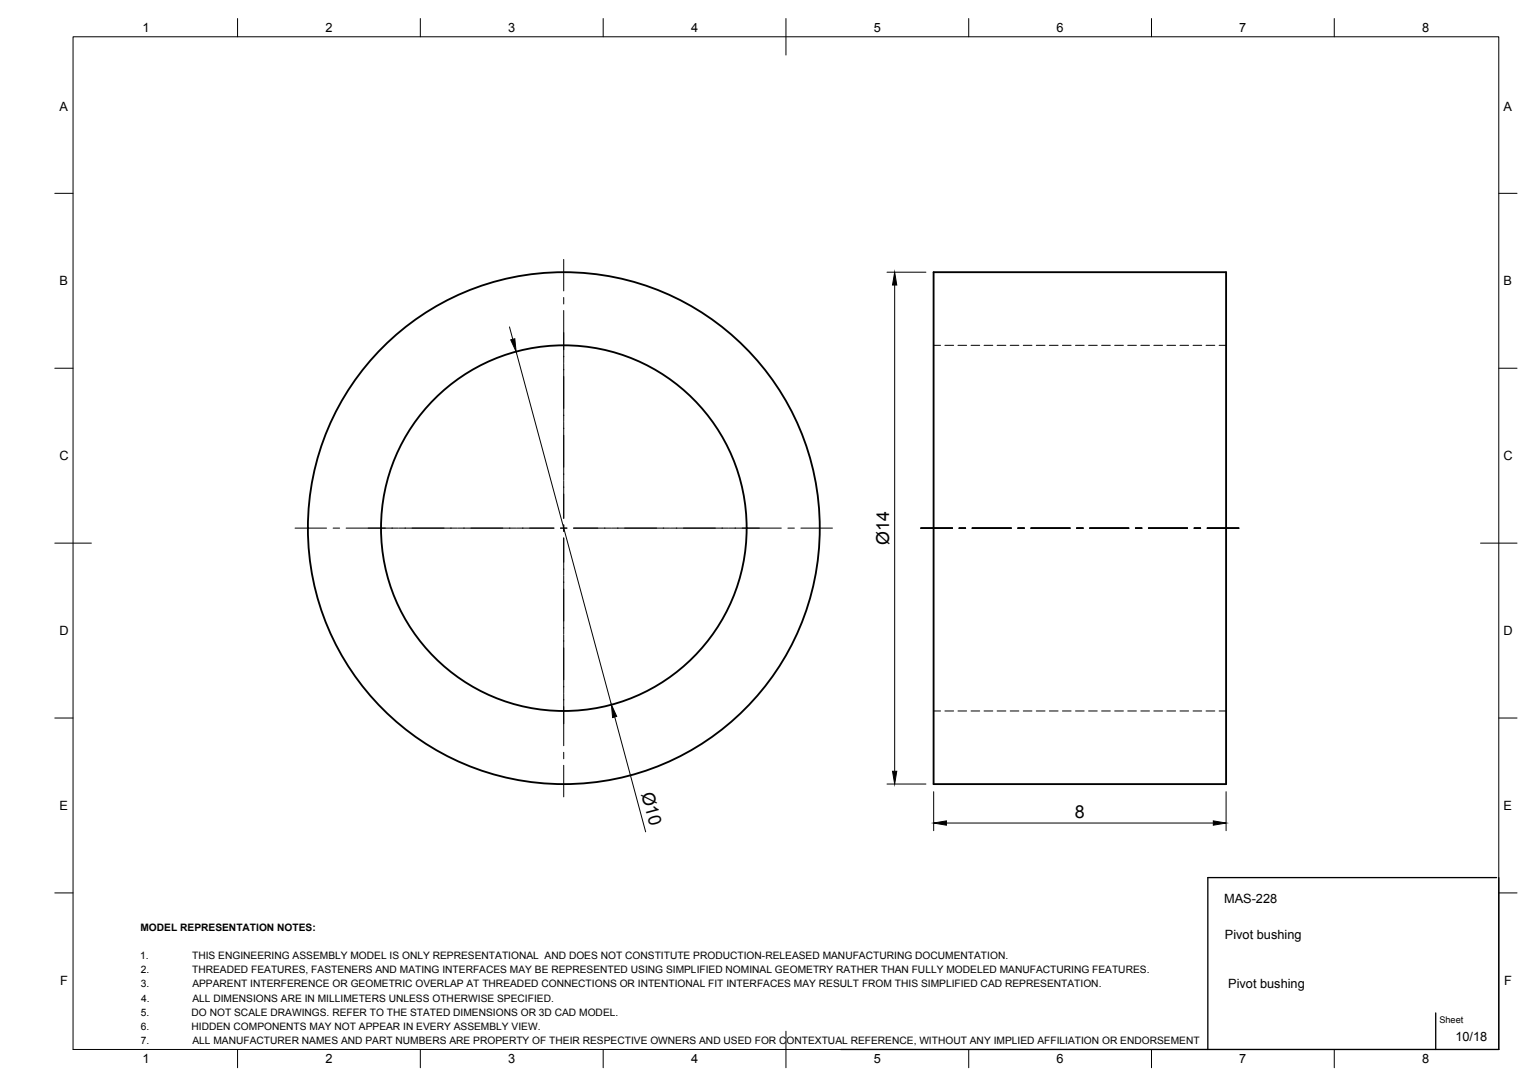
ISO-10303-21;
HEADER;
/* Generated by software containing ST-Developer
 * from STEP Tools, Inc. (www.steptools.com) 
 */

FILE_DESCRIPTION(
/* description */ ('Independent Peaucellier-Lipkin straight-line linkage. Radius arms 100
 mm, inversion-cell links 60 mm, crank radius and fixed-pivot spacing 
32 mm. Inversion constant 6400 mm squared, nominal output straight lin
e X=100 mm. Overhead bearing bridge clears the layered moving links. N
o accuracy or load rating assigned.'),
/* implementation_level */ '2;1');

FILE_NAME(
/* name */ 'Pivot bushing.step',
/* time_stamp */ '2026-11-09T18:06:16-08:00',
/* author */ (''),
/* organization */ (''),
/* preprocessor_version */ 'ST-DEVELOPER v20.2',
/* originating_system */ 'Autodesk Translation Framework v15.17.0.0',
/* authorisation */ '');

FILE_SCHEMA (('AUTOMOTIVE_DESIGN { 1 0 10303 214 3 1 1 }'));
ENDSEC;

DATA;
#10=MECHANICAL_DESIGN_GEOMETRIC_PRESENTATION_REPRESENTATION('',(#293),#3581);
#259=SHAPE_REPRESENTATION_RELATIONSHIP('SRR','None',#3693,#276);
#276=ADVANCED_BREP_SHAPE_REPRESENTATION('',(#310),#3575);
#293=STYLED_ITEM('',(#3784),#310);
#310=MANIFOLD_SOLID_BREP('Body1',#1879);
#355=FACE_BOUND('',#659,.T.);
#356=FACE_BOUND('',#661,.T.);
#409=PLANE('',#2245);
#410=PLANE('',#2246);
#506=FACE_OUTER_BOUND('',#656,.T.);
#507=FACE_OUTER_BOUND('',#657,.T.);
#508=FACE_OUTER_BOUND('',#658,.T.);
#509=FACE_OUTER_BOUND('',#660,.T.);
#656=EDGE_LOOP('',(#1616,#1617,#1618,#1619));
#657=EDGE_LOOP('',(#1620,#1621,#1622,#1623));
#658=EDGE_LOOP('',(#1624));
#659=EDGE_LOOP('',(#1625));
#660=EDGE_LOOP('',(#1626));
#661=EDGE_LOOP('',(#1627));
#773=LINE('',#3377,#871);
#774=LINE('',#3383,#872);
#871=VECTOR('',#2773,5.);
#872=VECTOR('',#2780,7.);
#963=CIRCLE('',#2240,5.);
#964=CIRCLE('',#2241,5.);
#965=CIRCLE('',#2243,7.);
#966=CIRCLE('',#2244,7.);
#1089=VERTEX_POINT('',#3374);
#1090=VERTEX_POINT('',#3376);
#1091=VERTEX_POINT('',#3380);
#1092=VERTEX_POINT('',#3382);
#1270=EDGE_CURVE('',#1089,#1089,#963,.T.);
#1271=EDGE_CURVE('',#1089,#1090,#773,.T.);
#1272=EDGE_CURVE('',#1090,#1090,#964,.T.);
#1273=EDGE_CURVE('',#1091,#1091,#965,.T.);
#1274=EDGE_CURVE('',#1091,#1092,#774,.T.);
#1275=EDGE_CURVE('',#1092,#1092,#966,.T.);
#1616=ORIENTED_EDGE('',*,*,#1270,.F.);
#1617=ORIENTED_EDGE('',*,*,#1271,.T.);
#1618=ORIENTED_EDGE('',*,*,#1272,.T.);
#1619=ORIENTED_EDGE('',*,*,#1271,.F.);
#1620=ORIENTED_EDGE('',*,*,#1273,.F.);
#1621=ORIENTED_EDGE('',*,*,#1274,.T.);
#1622=ORIENTED_EDGE('',*,*,#1275,.T.);
#1623=ORIENTED_EDGE('',*,*,#1274,.F.);
#1624=ORIENTED_EDGE('',*,*,#1273,.T.);
#1625=ORIENTED_EDGE('',*,*,#1270,.T.);
#1626=ORIENTED_EDGE('',*,*,#1275,.F.);
#1627=ORIENTED_EDGE('',*,*,#1272,.F.);
#1744=CYLINDRICAL_SURFACE('',#2239,5.);
#1745=CYLINDRICAL_SURFACE('',#2242,7.);
#1838=ADVANCED_FACE('',(#506),#1744,.F.);
#1839=ADVANCED_FACE('',(#507),#1745,.T.);
#1840=ADVANCED_FACE('',(#508,#355),#409,.T.);
#1841=ADVANCED_FACE('',(#509,#356),#410,.F.);
#1879=CLOSED_SHELL('',(#1838,#1839,#1840,#1841));
#2238=AXIS2_PLACEMENT_3D('',#3372,#2767,#2768);
#2239=AXIS2_PLACEMENT_3D('',#3373,#2769,#2770);
#2240=AXIS2_PLACEMENT_3D('',#3375,#2771,#2772);
#2241=AXIS2_PLACEMENT_3D('',#3378,#2774,#2775);
#2242=AXIS2_PLACEMENT_3D('',#3379,#2776,#2777);
#2243=AXIS2_PLACEMENT_3D('',#3381,#2778,#2779);
#2244=AXIS2_PLACEMENT_3D('',#3384,#2781,#2782);
#2245=AXIS2_PLACEMENT_3D('',#3385,#2783,#2784);
#2246=AXIS2_PLACEMENT_3D('',#3386,#2785,#2786);
#2767=DIRECTION('axis',(0.,0.,1.));
#2768=DIRECTION('refdir',(1.,0.,0.));
#2769=DIRECTION('center_axis',(0.,0.,1.));
#2770=DIRECTION('ref_axis',(1.,0.,0.));
#2771=DIRECTION('center_axis',(0.,0.,-1.));
#2772=DIRECTION('ref_axis',(1.,0.,0.));
#2773=DIRECTION('',(0.,0.,-1.));
#2774=DIRECTION('center_axis',(0.,0.,-1.));
#2775=DIRECTION('ref_axis',(1.,0.,0.));
#2776=DIRECTION('center_axis',(0.,0.,1.));
#2777=DIRECTION('ref_axis',(1.,0.,0.));
#2778=DIRECTION('center_axis',(0.,0.,1.));
#2779=DIRECTION('ref_axis',(1.,0.,0.));
#2780=DIRECTION('',(0.,0.,-1.));
#2781=DIRECTION('center_axis',(0.,0.,1.));
#2782=DIRECTION('ref_axis',(1.,0.,0.));
#2783=DIRECTION('center_axis',(0.,0.,1.));
#2784=DIRECTION('ref_axis',(1.,0.,0.));
#2785=DIRECTION('center_axis',(0.,0.,1.));
#2786=DIRECTION('ref_axis',(1.,0.,0.));
#3372=CARTESIAN_POINT('',(0.,0.,0.));
#3373=CARTESIAN_POINT('Origin',(0.,0.,0.));
#3374=CARTESIAN_POINT('',(-5.,-6.12323399573677E-16,8.));
#3375=CARTESIAN_POINT('Origin',(0.,0.,8.));
#3376=CARTESIAN_POINT('',(-5.,-6.12323399573677E-16,0.));
#3377=CARTESIAN_POINT('',(-5.,-6.12323399573677E-16,0.));
#3378=CARTESIAN_POINT('Origin',(0.,0.,0.));
#3379=CARTESIAN_POINT('Origin',(0.,0.,0.));
#3380=CARTESIAN_POINT('',(-7.,-8.57252759403147E-16,8.));
#3381=CARTESIAN_POINT('Origin',(0.,0.,8.));
#3382=CARTESIAN_POINT('',(-7.,-8.57252759403147E-16,0.));
#3383=CARTESIAN_POINT('',(-7.,-8.57252759403147E-16,0.));
#3384=CARTESIAN_POINT('Origin',(0.,0.,0.));
#3385=CARTESIAN_POINT('Origin',(0.,0.,8.));
#3386=CARTESIAN_POINT('Origin',(0.,0.,0.));
#3556=UNCERTAINTY_MEASURE_WITH_UNIT(LENGTH_MEASURE(0.01),#3582,
'DISTANCE_ACCURACY_VALUE',
'Maximum model space distance between geometric entities at asserted c
onnectivities');
#3562=UNCERTAINTY_MEASURE_WITH_UNIT(LENGTH_MEASURE(0.01),#3582,
'DISTANCE_ACCURACY_VALUE',
'Maximum model space distance between geometric entities at asserted c
onnectivities');
#3575=(
GEOMETRIC_REPRESENTATION_CONTEXT(3)
GLOBAL_UNCERTAINTY_ASSIGNED_CONTEXT((#3556))
GLOBAL_UNIT_ASSIGNED_CONTEXT((#3582,#3584,#3585))
REPRESENTATION_CONTEXT('','3D')
);
#3581=(
GEOMETRIC_REPRESENTATION_CONTEXT(3)
GLOBAL_UNCERTAINTY_ASSIGNED_CONTEXT((#3562))
GLOBAL_UNIT_ASSIGNED_CONTEXT((#3582,#3584,#3585))
REPRESENTATION_CONTEXT('','3D')
);
#3582=(
LENGTH_UNIT()
NAMED_UNIT(*)
SI_UNIT(.MILLI.,.METRE.)
);
#3584=(
NAMED_UNIT(*)
PLANE_ANGLE_UNIT()
SI_UNIT($,.RADIAN.)
);
#3585=(
NAMED_UNIT(*)
SI_UNIT($,.STERADIAN.)
SOLID_ANGLE_UNIT()
);
#3598=SHAPE_DEFINITION_REPRESENTATION(#3616,#3693);
#3616=PRODUCT_DEFINITION_SHAPE('',$,#3712);
#3693=SHAPE_REPRESENTATION('',(#2238),#3575);
#3699=PRODUCT_DEFINITION_CONTEXT('part definition',#3755,'design');
#3712=PRODUCT_DEFINITION('Pivot bushing','Pivot bushing',#3730,#3699);
#3730=PRODUCT_DEFINITION_FORMATION('',$,#3769);
#3755=APPLICATION_CONTEXT(
'Core Data for Automotive Mechanical Design Process');
#3756=PRODUCT_CONTEXT('part definition',#3755,'mechanical');
#3769=PRODUCT('Pivot bushing','Pivot bushing',$,(#3756));
#3784=PRESENTATION_STYLE_ASSIGNMENT((#3797));
#3797=SURFACE_STYLE_USAGE(.BOTH.,#3810);
#3810=SURFACE_SIDE_STYLE('',(#3823));
#3823=SURFACE_STYLE_FILL_AREA(#3836);
#3836=FILL_AREA_STYLE('Bearing light gray',(#3849));
#3849=FILL_AREA_STYLE_COLOUR('Bearing light gray',#3862);
#3862=COLOUR_RGB('Bearing light gray',0.725490196078431,0.752941176470588,
0.792156862745098);
ENDSEC;
END-ISO-10303-21;
